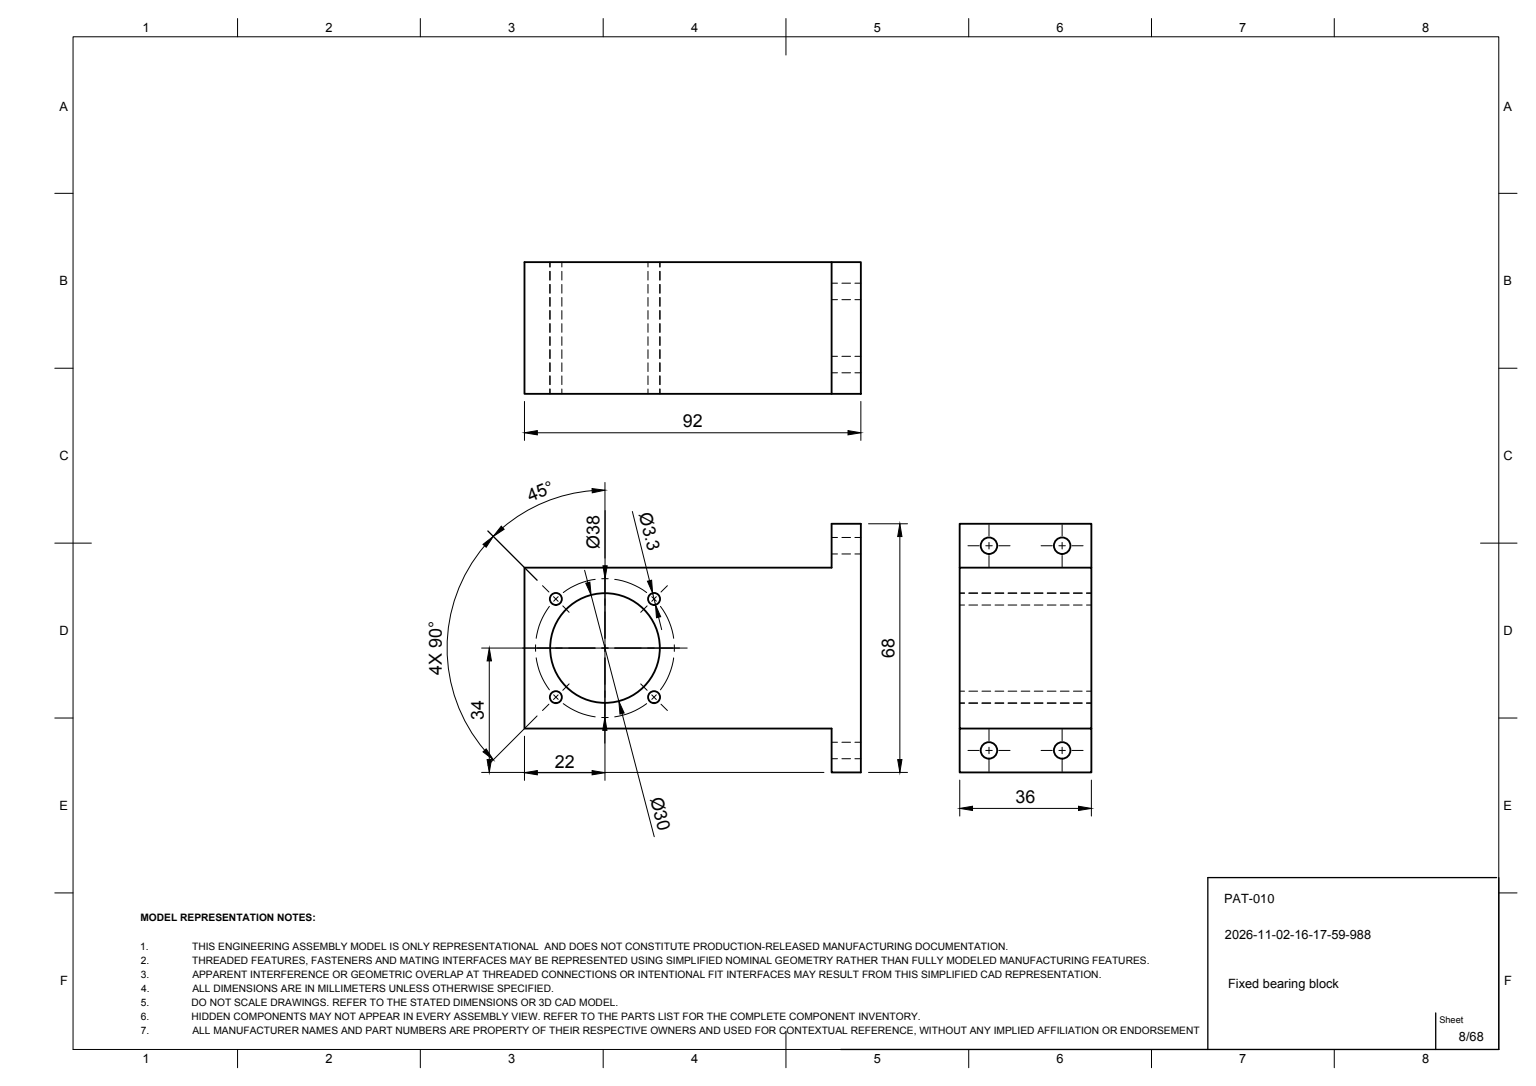
ISO-10303-21;
HEADER;
/* Generated by software containing ST-Developer
 * from STEP Tools, Inc. (www.steptools.com) 
 */

FILE_DESCRIPTION(
/* description */ ('Belt conveyor head drive unit'),
/* implementation_level */ '2;1');

FILE_NAME(
/* name */ 'Fixed bearing block.step',
/* time_stamp */ '2026-10-28T03:26:19-07:00',
/* author */ (''),
/* organization */ (''),
/* preprocessor_version */ 'ST-DEVELOPER v20.2',
/* originating_system */ 'Autodesk Translation Framework v15.17.0.0',
/* authorisation */ '');

FILE_SCHEMA (('AUTOMOTIVE_DESIGN { 1 0 10303 214 3 1 1 }'));
ENDSEC;

DATA;
#10=MECHANICAL_DESIGN_GEOMETRIC_PRESENTATION_REPRESENTATION('',(#850),#27069);
#712=SHAPE_REPRESENTATION_RELATIONSHIP('SRR','None',#27356,#781);
#781=ADVANCED_BREP_SHAPE_REPRESENTATION('',(#935),#26998);
#850=STYLED_ITEM('',(#27797),#935);
#935=MANIFOLD_SOLID_BREP('Body1',#13715);
#1032=FACE_BOUND('',#2525,.T.);
#1033=FACE_BOUND('',#2526,.T.);
#1034=FACE_BOUND('',#2528,.T.);
#1035=FACE_BOUND('',#2529,.T.);
#1036=FACE_BOUND('',#2533,.T.);
#1037=FACE_BOUND('',#2534,.T.);
#1038=FACE_BOUND('',#2535,.T.);
#1039=FACE_BOUND('',#2536,.T.);
#1040=FACE_BOUND('',#2537,.T.);
#1041=FACE_BOUND('',#2540,.T.);
#1042=FACE_BOUND('',#2541,.T.);
#1043=FACE_BOUND('',#2542,.T.);
#1044=FACE_BOUND('',#2543,.T.);
#1045=FACE_BOUND('',#2544,.T.);
#1046=FACE_BOUND('',#2548,.T.);
#1047=FACE_BOUND('',#2549,.T.);
#1048=FACE_BOUND('',#2550,.T.);
#1049=FACE_BOUND('',#2551,.T.);
#1317=PLANE('',#14705);
#1318=PLANE('',#14706);
#1319=PLANE('',#14707);
#1320=PLANE('',#14708);
#1321=PLANE('',#14709);
#1322=PLANE('',#14710);
#1323=PLANE('',#14711);
#1324=PLANE('',#14712);
#1325=PLANE('',#14713);
#1326=PLANE('',#14714);
#1695=FACE_OUTER_BOUND('',#2515,.T.);
#1696=FACE_OUTER_BOUND('',#2516,.T.);
#1697=FACE_OUTER_BOUND('',#2517,.T.);
#1698=FACE_OUTER_BOUND('',#2518,.T.);
#1699=FACE_OUTER_BOUND('',#2519,.T.);
#1700=FACE_OUTER_BOUND('',#2520,.T.);
#1701=FACE_OUTER_BOUND('',#2521,.T.);
#1702=FACE_OUTER_BOUND('',#2522,.T.);
#1703=FACE_OUTER_BOUND('',#2523,.T.);
#1704=FACE_OUTER_BOUND('',#2524,.T.);
#1705=FACE_OUTER_BOUND('',#2527,.T.);
#1706=FACE_OUTER_BOUND('',#2530,.T.);
#1707=FACE_OUTER_BOUND('',#2531,.T.);
#1708=FACE_OUTER_BOUND('',#2532,.T.);
#1709=FACE_OUTER_BOUND('',#2538,.T.);
#1710=FACE_OUTER_BOUND('',#2539,.T.);
#1711=FACE_OUTER_BOUND('',#2545,.T.);
#1712=FACE_OUTER_BOUND('',#2546,.T.);
#1713=FACE_OUTER_BOUND('',#2547,.T.);
#2515=EDGE_LOOP('',(#9222,#9223,#9224,#9225));
#2516=EDGE_LOOP('',(#9226,#9227,#9228,#9229));
#2517=EDGE_LOOP('',(#9230,#9231,#9232,#9233));
#2518=EDGE_LOOP('',(#9234,#9235,#9236,#9237));
#2519=EDGE_LOOP('',(#9238,#9239,#9240,#9241));
#2520=EDGE_LOOP('',(#9242,#9243,#9244,#9245));
#2521=EDGE_LOOP('',(#9246,#9247,#9248,#9249));
#2522=EDGE_LOOP('',(#9250,#9251,#9252,#9253));
#2523=EDGE_LOOP('',(#9254,#9255,#9256,#9257));
#2524=EDGE_LOOP('',(#9258,#9259,#9260,#9261));
#2525=EDGE_LOOP('',(#9262));
#2526=EDGE_LOOP('',(#9263));
#2527=EDGE_LOOP('',(#9264,#9265,#9266,#9267));
#2528=EDGE_LOOP('',(#9268));
#2529=EDGE_LOOP('',(#9269));
#2530=EDGE_LOOP('',(#9270,#9271,#9272,#9273));
#2531=EDGE_LOOP('',(#9274,#9275,#9276,#9277));
#2532=EDGE_LOOP('',(#9278,#9279,#9280,#9281,#9282,#9283,#9284,#9285));
#2533=EDGE_LOOP('',(#9286));
#2534=EDGE_LOOP('',(#9287));
#2535=EDGE_LOOP('',(#9288));
#2536=EDGE_LOOP('',(#9289));
#2537=EDGE_LOOP('',(#9290));
#2538=EDGE_LOOP('',(#9291,#9292,#9293,#9294));
#2539=EDGE_LOOP('',(#9295,#9296,#9297,#9298,#9299,#9300,#9301,#9302));
#2540=EDGE_LOOP('',(#9303));
#2541=EDGE_LOOP('',(#9304));
#2542=EDGE_LOOP('',(#9305));
#2543=EDGE_LOOP('',(#9306));
#2544=EDGE_LOOP('',(#9307));
#2545=EDGE_LOOP('',(#9308,#9309,#9310,#9311));
#2546=EDGE_LOOP('',(#9312,#9313,#9314,#9315));
#2547=EDGE_LOOP('',(#9316,#9317,#9318,#9319));
#2548=EDGE_LOOP('',(#9320));
#2549=EDGE_LOOP('',(#9321));
#2550=EDGE_LOOP('',(#9322));
#2551=EDGE_LOOP('',(#9323));
#3582=LINE('',#21262,#4374);
#3583=LINE('',#21268,#4375);
#3584=LINE('',#21274,#4376);
#3585=LINE('',#21280,#4377);
#3586=LINE('',#21286,#4378);
#3587=LINE('',#21292,#4379);
#3588=LINE('',#21298,#4380);
#3589=LINE('',#21304,#4381);
#3590=LINE('',#21310,#4382);
#3591=LINE('',#21315,#4383);
#3592=LINE('',#21317,#4384);
#3593=LINE('',#21319,#4385);
#3594=LINE('',#21320,#4386);
#3595=LINE('',#21324,#4387);
#3596=LINE('',#21326,#4388);
#3597=LINE('',#21328,#4389);
#3598=LINE('',#21329,#4390);
#3599=LINE('',#21332,#4391);
#3600=LINE('',#21334,#4392);
#3601=LINE('',#21335,#4393);
#3602=LINE('',#21338,#4394);
#3603=LINE('',#21340,#4395);
#3604=LINE('',#21341,#4396);
#3605=LINE('',#21344,#4397);
#3606=LINE('',#21346,#4398);
#3607=LINE('',#21347,#4399);
#3608=LINE('',#21348,#4400);
#3609=LINE('',#21351,#4401);
#3610=LINE('',#21352,#4402);
#3611=LINE('',#21355,#4403);
#3612=LINE('',#21356,#4404);
#3613=LINE('',#21357,#4405);
#3614=LINE('',#21359,#4406);
#4374=VECTOR('',#16754,0.165);
#4375=VECTOR('',#16761,0.165);
#4376=VECTOR('',#16768,0.165);
#4377=VECTOR('',#16775,0.165);
#4378=VECTOR('',#16782,1.5);
#4379=VECTOR('',#16789,0.225);
#4380=VECTOR('',#16796,0.225);
#4381=VECTOR('',#16803,0.225);
#4382=VECTOR('',#16810,0.225);
#4383=VECTOR('',#16815,1.);
#4384=VECTOR('',#16816,1.);
#4385=VECTOR('',#16817,1.);
#4386=VECTOR('',#16818,1.);
#4387=VECTOR('',#16821,1.);
#4388=VECTOR('',#16822,1.);
#4389=VECTOR('',#16823,1.);
#4390=VECTOR('',#16824,1.);
#4391=VECTOR('',#16827,1.);
#4392=VECTOR('',#16828,1.);
#4393=VECTOR('',#16829,1.);
#4394=VECTOR('',#16832,1.);
#4395=VECTOR('',#16833,1.);
#4396=VECTOR('',#16834,1.);
#4397=VECTOR('',#16837,1.);
#4398=VECTOR('',#16838,1.);
#4399=VECTOR('',#16839,1.);
#4400=VECTOR('',#16840,1.);
#4401=VECTOR('',#16843,1.);
#4402=VECTOR('',#16844,1.);
#4403=VECTOR('',#16847,1.);
#4404=VECTOR('',#16848,1.);
#4405=VECTOR('',#16849,1.);
#4406=VECTOR('',#16852,1.);
#5130=CIRCLE('',#14679,0.165);
#5131=CIRCLE('',#14680,0.165);
#5132=CIRCLE('',#14682,0.165);
#5133=CIRCLE('',#14683,0.165);
#5134=CIRCLE('',#14685,0.165);
#5135=CIRCLE('',#14686,0.165);
#5136=CIRCLE('',#14688,0.165);
#5137=CIRCLE('',#14689,0.165);
#5138=CIRCLE('',#14691,1.5);
#5139=CIRCLE('',#14692,1.5);
#5140=CIRCLE('',#14694,0.225);
#5141=CIRCLE('',#14695,0.225);
#5142=CIRCLE('',#14697,0.225);
#5143=CIRCLE('',#14698,0.225);
#5144=CIRCLE('',#14700,0.225);
#5145=CIRCLE('',#14701,0.225);
#5146=CIRCLE('',#14703,0.225);
#5147=CIRCLE('',#14704,0.225);
#6041=VERTEX_POINT('',#21259);
#6042=VERTEX_POINT('',#21261);
#6043=VERTEX_POINT('',#21265);
#6044=VERTEX_POINT('',#21267);
#6045=VERTEX_POINT('',#21271);
#6046=VERTEX_POINT('',#21273);
#6047=VERTEX_POINT('',#21277);
#6048=VERTEX_POINT('',#21279);
#6049=VERTEX_POINT('',#21283);
#6050=VERTEX_POINT('',#21285);
#6051=VERTEX_POINT('',#21289);
#6052=VERTEX_POINT('',#21291);
#6053=VERTEX_POINT('',#21295);
#6054=VERTEX_POINT('',#21297);
#6055=VERTEX_POINT('',#21301);
#6056=VERTEX_POINT('',#21303);
#6057=VERTEX_POINT('',#21307);
#6058=VERTEX_POINT('',#21309);
#6059=VERTEX_POINT('',#21313);
#6060=VERTEX_POINT('',#21314);
#6061=VERTEX_POINT('',#21316);
#6062=VERTEX_POINT('',#21318);
#6063=VERTEX_POINT('',#21322);
#6064=VERTEX_POINT('',#21323);
#6065=VERTEX_POINT('',#21325);
#6066=VERTEX_POINT('',#21327);
#6067=VERTEX_POINT('',#21331);
#6068=VERTEX_POINT('',#21333);
#6069=VERTEX_POINT('',#21337);
#6070=VERTEX_POINT('',#21339);
#6071=VERTEX_POINT('',#21343);
#6072=VERTEX_POINT('',#21345);
#6073=VERTEX_POINT('',#21350);
#6074=VERTEX_POINT('',#21354);
#7303=EDGE_CURVE('',#6041,#6041,#5130,.T.);
#7304=EDGE_CURVE('',#6041,#6042,#3582,.T.);
#7305=EDGE_CURVE('',#6042,#6042,#5131,.T.);
#7306=EDGE_CURVE('',#6043,#6043,#5132,.T.);
#7307=EDGE_CURVE('',#6043,#6044,#3583,.T.);
#7308=EDGE_CURVE('',#6044,#6044,#5133,.T.);
#7309=EDGE_CURVE('',#6045,#6045,#5134,.T.);
#7310=EDGE_CURVE('',#6045,#6046,#3584,.T.);
#7311=EDGE_CURVE('',#6046,#6046,#5135,.T.);
#7312=EDGE_CURVE('',#6047,#6047,#5136,.T.);
#7313=EDGE_CURVE('',#6047,#6048,#3585,.T.);
#7314=EDGE_CURVE('',#6048,#6048,#5137,.T.);
#7315=EDGE_CURVE('',#6049,#6049,#5138,.T.);
#7316=EDGE_CURVE('',#6049,#6050,#3586,.T.);
#7317=EDGE_CURVE('',#6050,#6050,#5139,.T.);
#7318=EDGE_CURVE('',#6051,#6051,#5140,.T.);
#7319=EDGE_CURVE('',#6051,#6052,#3587,.T.);
#7320=EDGE_CURVE('',#6052,#6052,#5141,.T.);
#7321=EDGE_CURVE('',#6053,#6053,#5142,.T.);
#7322=EDGE_CURVE('',#6053,#6054,#3588,.T.);
#7323=EDGE_CURVE('',#6054,#6054,#5143,.T.);
#7324=EDGE_CURVE('',#6055,#6055,#5144,.T.);
#7325=EDGE_CURVE('',#6055,#6056,#3589,.T.);
#7326=EDGE_CURVE('',#6056,#6056,#5145,.T.);
#7327=EDGE_CURVE('',#6057,#6057,#5146,.T.);
#7328=EDGE_CURVE('',#6057,#6058,#3590,.T.);
#7329=EDGE_CURVE('',#6058,#6058,#5147,.T.);
#7330=EDGE_CURVE('',#6059,#6060,#3591,.T.);
#7331=EDGE_CURVE('',#6061,#6059,#3592,.T.);
#7332=EDGE_CURVE('',#6061,#6062,#3593,.T.);
#7333=EDGE_CURVE('',#6060,#6062,#3594,.T.);
#7334=EDGE_CURVE('',#6063,#6064,#3595,.T.);
#7335=EDGE_CURVE('',#6065,#6063,#3596,.T.);
#7336=EDGE_CURVE('',#6066,#6065,#3597,.T.);
#7337=EDGE_CURVE('',#6064,#6066,#3598,.T.);
#7338=EDGE_CURVE('',#6066,#6067,#3599,.T.);
#7339=EDGE_CURVE('',#6068,#6065,#3600,.T.);
#7340=EDGE_CURVE('',#6067,#6068,#3601,.T.);
#7341=EDGE_CURVE('',#6069,#6061,#3602,.T.);
#7342=EDGE_CURVE('',#6069,#6070,#3603,.T.);
#7343=EDGE_CURVE('',#6062,#6070,#3604,.T.);
#7344=EDGE_CURVE('',#6059,#6071,#3605,.T.);
#7345=EDGE_CURVE('',#6072,#6071,#3606,.T.);
#7346=EDGE_CURVE('',#6064,#6072,#3607,.T.);
#7347=EDGE_CURVE('',#6067,#6069,#3608,.T.);
#7348=EDGE_CURVE('',#6060,#6073,#3609,.T.);
#7349=EDGE_CURVE('',#6071,#6073,#3610,.T.);
#7350=EDGE_CURVE('',#6063,#6074,#3611,.T.);
#7351=EDGE_CURVE('',#6073,#6074,#3612,.T.);
#7352=EDGE_CURVE('',#6070,#6068,#3613,.T.);
#7353=EDGE_CURVE('',#6074,#6072,#3614,.T.);
#9222=ORIENTED_EDGE('',*,*,#7303,.F.);
#9223=ORIENTED_EDGE('',*,*,#7304,.T.);
#9224=ORIENTED_EDGE('',*,*,#7305,.F.);
#9225=ORIENTED_EDGE('',*,*,#7304,.F.);
#9226=ORIENTED_EDGE('',*,*,#7306,.F.);
#9227=ORIENTED_EDGE('',*,*,#7307,.T.);
#9228=ORIENTED_EDGE('',*,*,#7308,.F.);
#9229=ORIENTED_EDGE('',*,*,#7307,.F.);
#9230=ORIENTED_EDGE('',*,*,#7309,.F.);
#9231=ORIENTED_EDGE('',*,*,#7310,.T.);
#9232=ORIENTED_EDGE('',*,*,#7311,.F.);
#9233=ORIENTED_EDGE('',*,*,#7310,.F.);
#9234=ORIENTED_EDGE('',*,*,#7312,.F.);
#9235=ORIENTED_EDGE('',*,*,#7313,.T.);
#9236=ORIENTED_EDGE('',*,*,#7314,.F.);
#9237=ORIENTED_EDGE('',*,*,#7313,.F.);
#9238=ORIENTED_EDGE('',*,*,#7315,.F.);
#9239=ORIENTED_EDGE('',*,*,#7316,.T.);
#9240=ORIENTED_EDGE('',*,*,#7317,.F.);
#9241=ORIENTED_EDGE('',*,*,#7316,.F.);
#9242=ORIENTED_EDGE('',*,*,#7318,.F.);
#9243=ORIENTED_EDGE('',*,*,#7319,.T.);
#9244=ORIENTED_EDGE('',*,*,#7320,.F.);
#9245=ORIENTED_EDGE('',*,*,#7319,.F.);
#9246=ORIENTED_EDGE('',*,*,#7321,.F.);
#9247=ORIENTED_EDGE('',*,*,#7322,.T.);
#9248=ORIENTED_EDGE('',*,*,#7323,.F.);
#9249=ORIENTED_EDGE('',*,*,#7322,.F.);
#9250=ORIENTED_EDGE('',*,*,#7324,.F.);
#9251=ORIENTED_EDGE('',*,*,#7325,.T.);
#9252=ORIENTED_EDGE('',*,*,#7326,.F.);
#9253=ORIENTED_EDGE('',*,*,#7325,.F.);
#9254=ORIENTED_EDGE('',*,*,#7327,.F.);
#9255=ORIENTED_EDGE('',*,*,#7328,.T.);
#9256=ORIENTED_EDGE('',*,*,#7329,.F.);
#9257=ORIENTED_EDGE('',*,*,#7328,.F.);
#9258=ORIENTED_EDGE('',*,*,#7330,.F.);
#9259=ORIENTED_EDGE('',*,*,#7331,.F.);
#9260=ORIENTED_EDGE('',*,*,#7332,.T.);
#9261=ORIENTED_EDGE('',*,*,#7333,.F.);
#9262=ORIENTED_EDGE('',*,*,#7320,.T.);
#9263=ORIENTED_EDGE('',*,*,#7329,.T.);
#9264=ORIENTED_EDGE('',*,*,#7334,.F.);
#9265=ORIENTED_EDGE('',*,*,#7335,.F.);
#9266=ORIENTED_EDGE('',*,*,#7336,.F.);
#9267=ORIENTED_EDGE('',*,*,#7337,.F.);
#9268=ORIENTED_EDGE('',*,*,#7323,.T.);
#9269=ORIENTED_EDGE('',*,*,#7326,.T.);
#9270=ORIENTED_EDGE('',*,*,#7338,.F.);
#9271=ORIENTED_EDGE('',*,*,#7336,.T.);
#9272=ORIENTED_EDGE('',*,*,#7339,.F.);
#9273=ORIENTED_EDGE('',*,*,#7340,.F.);
#9274=ORIENTED_EDGE('',*,*,#7341,.F.);
#9275=ORIENTED_EDGE('',*,*,#7342,.T.);
#9276=ORIENTED_EDGE('',*,*,#7343,.F.);
#9277=ORIENTED_EDGE('',*,*,#7332,.F.);
#9278=ORIENTED_EDGE('',*,*,#7344,.T.);
#9279=ORIENTED_EDGE('',*,*,#7345,.F.);
#9280=ORIENTED_EDGE('',*,*,#7346,.F.);
#9281=ORIENTED_EDGE('',*,*,#7337,.T.);
#9282=ORIENTED_EDGE('',*,*,#7338,.T.);
#9283=ORIENTED_EDGE('',*,*,#7347,.T.);
#9284=ORIENTED_EDGE('',*,*,#7341,.T.);
#9285=ORIENTED_EDGE('',*,*,#7331,.T.);
#9286=ORIENTED_EDGE('',*,*,#7315,.T.);
#9287=ORIENTED_EDGE('',*,*,#7312,.T.);
#9288=ORIENTED_EDGE('',*,*,#7309,.T.);
#9289=ORIENTED_EDGE('',*,*,#7306,.T.);
#9290=ORIENTED_EDGE('',*,*,#7303,.T.);
#9291=ORIENTED_EDGE('',*,*,#7330,.T.);
#9292=ORIENTED_EDGE('',*,*,#7348,.T.);
#9293=ORIENTED_EDGE('',*,*,#7349,.F.);
#9294=ORIENTED_EDGE('',*,*,#7344,.F.);
#9295=ORIENTED_EDGE('',*,*,#7350,.T.);
#9296=ORIENTED_EDGE('',*,*,#7351,.F.);
#9297=ORIENTED_EDGE('',*,*,#7348,.F.);
#9298=ORIENTED_EDGE('',*,*,#7333,.T.);
#9299=ORIENTED_EDGE('',*,*,#7343,.T.);
#9300=ORIENTED_EDGE('',*,*,#7352,.T.);
#9301=ORIENTED_EDGE('',*,*,#7339,.T.);
#9302=ORIENTED_EDGE('',*,*,#7335,.T.);
#9303=ORIENTED_EDGE('',*,*,#7317,.T.);
#9304=ORIENTED_EDGE('',*,*,#7314,.T.);
#9305=ORIENTED_EDGE('',*,*,#7311,.T.);
#9306=ORIENTED_EDGE('',*,*,#7308,.T.);
#9307=ORIENTED_EDGE('',*,*,#7305,.T.);
#9308=ORIENTED_EDGE('',*,*,#7334,.T.);
#9309=ORIENTED_EDGE('',*,*,#7346,.T.);
#9310=ORIENTED_EDGE('',*,*,#7353,.F.);
#9311=ORIENTED_EDGE('',*,*,#7350,.F.);
#9312=ORIENTED_EDGE('',*,*,#7353,.T.);
#9313=ORIENTED_EDGE('',*,*,#7345,.T.);
#9314=ORIENTED_EDGE('',*,*,#7349,.T.);
#9315=ORIENTED_EDGE('',*,*,#7351,.T.);
#9316=ORIENTED_EDGE('',*,*,#7352,.F.);
#9317=ORIENTED_EDGE('',*,*,#7342,.F.);
#9318=ORIENTED_EDGE('',*,*,#7347,.F.);
#9319=ORIENTED_EDGE('',*,*,#7340,.T.);
#9320=ORIENTED_EDGE('',*,*,#7318,.T.);
#9321=ORIENTED_EDGE('',*,*,#7321,.T.);
#9322=ORIENTED_EDGE('',*,*,#7324,.T.);
#9323=ORIENTED_EDGE('',*,*,#7327,.T.);
#12554=CYLINDRICAL_SURFACE('',#14678,0.165);
#12555=CYLINDRICAL_SURFACE('',#14681,0.165);
#12556=CYLINDRICAL_SURFACE('',#14684,0.165);
#12557=CYLINDRICAL_SURFACE('',#14687,0.165);
#12558=CYLINDRICAL_SURFACE('',#14690,1.5);
#12559=CYLINDRICAL_SURFACE('',#14693,0.225);
#12560=CYLINDRICAL_SURFACE('',#14696,0.225);
#12561=CYLINDRICAL_SURFACE('',#14699,0.225);
#12562=CYLINDRICAL_SURFACE('',#14702,0.225);
#12974=ADVANCED_FACE('',(#1695),#12554,.F.);
#12975=ADVANCED_FACE('',(#1696),#12555,.F.);
#12976=ADVANCED_FACE('',(#1697),#12556,.F.);
#12977=ADVANCED_FACE('',(#1698),#12557,.F.);
#12978=ADVANCED_FACE('',(#1699),#12558,.F.);
#12979=ADVANCED_FACE('',(#1700),#12559,.F.);
#12980=ADVANCED_FACE('',(#1701),#12560,.F.);
#12981=ADVANCED_FACE('',(#1702),#12561,.F.);
#12982=ADVANCED_FACE('',(#1703),#12562,.F.);
#12983=ADVANCED_FACE('',(#1704,#1032,#1033),#1317,.T.);
#12984=ADVANCED_FACE('',(#1705,#1034,#1035),#1318,.T.);
#12985=ADVANCED_FACE('',(#1706),#1319,.T.);
#12986=ADVANCED_FACE('',(#1707),#1320,.T.);
#12987=ADVANCED_FACE('',(#1708,#1036,#1037,#1038,#1039,#1040),#1321,.T.);
#12988=ADVANCED_FACE('',(#1709),#1322,.T.);
#12989=ADVANCED_FACE('',(#1710,#1041,#1042,#1043,#1044,#1045),#1323,.T.);
#12990=ADVANCED_FACE('',(#1711),#1324,.T.);
#12991=ADVANCED_FACE('',(#1712),#1325,.T.);
#12992=ADVANCED_FACE('',(#1713,#1046,#1047,#1048,#1049),#1326,.F.);
#13715=CLOSED_SHELL('',(#12974,#12975,#12976,#12977,#12978,#12979,#12980,
#12981,#12982,#12983,#12984,#12985,#12986,#12987,#12988,#12989,#12990,#12991,
#12992));
#14677=AXIS2_PLACEMENT_3D('',#21257,#16748,#16749);
#14678=AXIS2_PLACEMENT_3D('',#21258,#16750,#16751);
#14679=AXIS2_PLACEMENT_3D('',#21260,#16752,#16753);
#14680=AXIS2_PLACEMENT_3D('',#21263,#16755,#16756);
#14681=AXIS2_PLACEMENT_3D('',#21264,#16757,#16758);
#14682=AXIS2_PLACEMENT_3D('',#21266,#16759,#16760);
#14683=AXIS2_PLACEMENT_3D('',#21269,#16762,#16763);
#14684=AXIS2_PLACEMENT_3D('',#21270,#16764,#16765);
#14685=AXIS2_PLACEMENT_3D('',#21272,#16766,#16767);
#14686=AXIS2_PLACEMENT_3D('',#21275,#16769,#16770);
#14687=AXIS2_PLACEMENT_3D('',#21276,#16771,#16772);
#14688=AXIS2_PLACEMENT_3D('',#21278,#16773,#16774);
#14689=AXIS2_PLACEMENT_3D('',#21281,#16776,#16777);
#14690=AXIS2_PLACEMENT_3D('',#21282,#16778,#16779);
#14691=AXIS2_PLACEMENT_3D('',#21284,#16780,#16781);
#14692=AXIS2_PLACEMENT_3D('',#21287,#16783,#16784);
#14693=AXIS2_PLACEMENT_3D('',#21288,#16785,#16786);
#14694=AXIS2_PLACEMENT_3D('',#21290,#16787,#16788);
#14695=AXIS2_PLACEMENT_3D('',#21293,#16790,#16791);
#14696=AXIS2_PLACEMENT_3D('',#21294,#16792,#16793);
#14697=AXIS2_PLACEMENT_3D('',#21296,#16794,#16795);
#14698=AXIS2_PLACEMENT_3D('',#21299,#16797,#16798);
#14699=AXIS2_PLACEMENT_3D('',#21300,#16799,#16800);
#14700=AXIS2_PLACEMENT_3D('',#21302,#16801,#16802);
#14701=AXIS2_PLACEMENT_3D('',#21305,#16804,#16805);
#14702=AXIS2_PLACEMENT_3D('',#21306,#16806,#16807);
#14703=AXIS2_PLACEMENT_3D('',#21308,#16808,#16809);
#14704=AXIS2_PLACEMENT_3D('',#21311,#16811,#16812);
#14705=AXIS2_PLACEMENT_3D('',#21312,#16813,#16814);
#14706=AXIS2_PLACEMENT_3D('',#21321,#16819,#16820);
#14707=AXIS2_PLACEMENT_3D('',#21330,#16825,#16826);
#14708=AXIS2_PLACEMENT_3D('',#21336,#16830,#16831);
#14709=AXIS2_PLACEMENT_3D('',#21342,#16835,#16836);
#14710=AXIS2_PLACEMENT_3D('',#21349,#16841,#16842);
#14711=AXIS2_PLACEMENT_3D('',#21353,#16845,#16846);
#14712=AXIS2_PLACEMENT_3D('',#21358,#16850,#16851);
#14713=AXIS2_PLACEMENT_3D('',#21360,#16853,#16854);
#14714=AXIS2_PLACEMENT_3D('',#21361,#16855,#16856);
#16748=DIRECTION('axis',(0.,0.,1.));
#16749=DIRECTION('refdir',(1.,0.,0.));
#16750=DIRECTION('center_axis',(0.,1.,0.));
#16751=DIRECTION('ref_axis',(1.,0.,0.));
#16752=DIRECTION('center_axis',(0.,1.,0.));
#16753=DIRECTION('ref_axis',(1.,0.,0.));
#16754=DIRECTION('',(0.,1.,0.));
#16755=DIRECTION('center_axis',(0.,-1.,0.));
#16756=DIRECTION('ref_axis',(1.,0.,0.));
#16757=DIRECTION('center_axis',(0.,1.,0.));
#16758=DIRECTION('ref_axis',(1.,0.,0.));
#16759=DIRECTION('center_axis',(0.,1.,0.));
#16760=DIRECTION('ref_axis',(1.,0.,0.));
#16761=DIRECTION('',(0.,1.,0.));
#16762=DIRECTION('center_axis',(0.,-1.,0.));
#16763=DIRECTION('ref_axis',(1.,0.,0.));
#16764=DIRECTION('center_axis',(0.,1.,0.));
#16765=DIRECTION('ref_axis',(1.,0.,0.));
#16766=DIRECTION('center_axis',(0.,1.,0.));
#16767=DIRECTION('ref_axis',(1.,0.,0.));
#16768=DIRECTION('',(0.,1.,0.));
#16769=DIRECTION('center_axis',(0.,-1.,0.));
#16770=DIRECTION('ref_axis',(1.,0.,0.));
#16771=DIRECTION('center_axis',(0.,1.,0.));
#16772=DIRECTION('ref_axis',(1.,0.,0.));
#16773=DIRECTION('center_axis',(0.,1.,0.));
#16774=DIRECTION('ref_axis',(1.,0.,0.));
#16775=DIRECTION('',(0.,1.,0.));
#16776=DIRECTION('center_axis',(0.,-1.,0.));
#16777=DIRECTION('ref_axis',(1.,0.,0.));
#16778=DIRECTION('center_axis',(0.,1.,0.));
#16779=DIRECTION('ref_axis',(1.,0.,0.));
#16780=DIRECTION('center_axis',(0.,1.,0.));
#16781=DIRECTION('ref_axis',(1.,0.,0.));
#16782=DIRECTION('',(0.,1.,0.));
#16783=DIRECTION('center_axis',(0.,-1.,0.));
#16784=DIRECTION('ref_axis',(1.,0.,0.));
#16785=DIRECTION('center_axis',(0.,0.,1.));
#16786=DIRECTION('ref_axis',(1.,0.,0.));
#16787=DIRECTION('center_axis',(0.,0.,1.));
#16788=DIRECTION('ref_axis',(1.,0.,0.));
#16789=DIRECTION('',(0.,0.,1.));
#16790=DIRECTION('center_axis',(0.,0.,-1.));
#16791=DIRECTION('ref_axis',(1.,0.,0.));
#16792=DIRECTION('center_axis',(0.,0.,1.));
#16793=DIRECTION('ref_axis',(1.,0.,0.));
#16794=DIRECTION('center_axis',(0.,0.,1.));
#16795=DIRECTION('ref_axis',(1.,0.,0.));
#16796=DIRECTION('',(0.,0.,1.));
#16797=DIRECTION('center_axis',(0.,0.,-1.));
#16798=DIRECTION('ref_axis',(1.,0.,0.));
#16799=DIRECTION('center_axis',(0.,0.,1.));
#16800=DIRECTION('ref_axis',(1.,0.,0.));
#16801=DIRECTION('center_axis',(0.,0.,1.));
#16802=DIRECTION('ref_axis',(1.,0.,0.));
#16803=DIRECTION('',(0.,0.,1.));
#16804=DIRECTION('center_axis',(0.,0.,-1.));
#16805=DIRECTION('ref_axis',(1.,0.,0.));
#16806=DIRECTION('center_axis',(0.,0.,1.));
#16807=DIRECTION('ref_axis',(1.,0.,0.));
#16808=DIRECTION('center_axis',(0.,0.,1.));
#16809=DIRECTION('ref_axis',(1.,0.,0.));
#16810=DIRECTION('',(0.,0.,1.));
#16811=DIRECTION('center_axis',(0.,0.,-1.));
#16812=DIRECTION('ref_axis',(1.,0.,0.));
#16813=DIRECTION('center_axis',(0.,0.,1.));
#16814=DIRECTION('ref_axis',(1.,0.,0.));
#16815=DIRECTION('',(0.,1.,0.));
#16816=DIRECTION('',(-1.,0.,0.));
#16817=DIRECTION('',(0.,1.,0.));
#16818=DIRECTION('',(1.,0.,0.));
#16819=DIRECTION('center_axis',(0.,0.,1.));
#16820=DIRECTION('ref_axis',(1.,0.,0.));
#16821=DIRECTION('',(0.,-1.,0.));
#16822=DIRECTION('',(1.,0.,0.));
#16823=DIRECTION('',(0.,1.,0.));
#16824=DIRECTION('',(-1.,0.,0.));
#16825=DIRECTION('center_axis',(-1.,0.,0.));
#16826=DIRECTION('ref_axis',(0.,0.,1.));
#16827=DIRECTION('',(0.,0.,-1.));
#16828=DIRECTION('',(0.,0.,1.));
#16829=DIRECTION('',(0.,1.,0.));
#16830=DIRECTION('center_axis',(1.,0.,0.));
#16831=DIRECTION('ref_axis',(0.,0.,-1.));
#16832=DIRECTION('',(0.,0.,1.));
#16833=DIRECTION('',(0.,1.,0.));
#16834=DIRECTION('',(0.,0.,-1.));
#16835=DIRECTION('center_axis',(0.,-1.,0.));
#16836=DIRECTION('ref_axis',(1.,0.,0.));
#16837=DIRECTION('',(0.,0.,1.));
#16838=DIRECTION('',(1.,0.,0.));
#16839=DIRECTION('',(0.,0.,1.));
#16840=DIRECTION('',(1.,0.,0.));
#16841=DIRECTION('center_axis',(1.,0.,0.));
#16842=DIRECTION('ref_axis',(0.,1.,0.));
#16843=DIRECTION('',(0.,0.,1.));
#16844=DIRECTION('',(0.,1.,0.));
#16845=DIRECTION('center_axis',(0.,1.,0.));
#16846=DIRECTION('ref_axis',(-1.,0.,0.));
#16847=DIRECTION('',(0.,0.,1.));
#16848=DIRECTION('',(-1.,0.,0.));
#16849=DIRECTION('',(-1.,0.,0.));
#16850=DIRECTION('center_axis',(-1.,0.,0.));
#16851=DIRECTION('ref_axis',(0.,-1.,0.));
#16852=DIRECTION('',(0.,-1.,0.));
#16853=DIRECTION('center_axis',(0.,0.,1.));
#16854=DIRECTION('ref_axis',(1.,0.,0.));
#16855=DIRECTION('center_axis',(0.,0.,1.));
#16856=DIRECTION('ref_axis',(1.,0.,0.));
#21257=CARTESIAN_POINT('',(0.,0.,0.));
#21258=CARTESIAN_POINT('Origin',(-1.34350288425444,-1.9,5.65649711574556));
#21259=CARTESIAN_POINT('',(-1.50850288425444,-1.8,5.65649711574556));
#21260=CARTESIAN_POINT('Origin',(-1.34350288425444,-1.8,5.65649711574556));
#21261=CARTESIAN_POINT('',(-1.50850288425444,1.8,5.65649711574556));
#21262=CARTESIAN_POINT('',(-1.50850288425444,-1.9,5.65649711574556));
#21263=CARTESIAN_POINT('Origin',(-1.34350288425444,1.8,5.65649711574556));
#21264=CARTESIAN_POINT('Origin',(-1.34350288425444,-1.9,8.34350288425444));
#21265=CARTESIAN_POINT('',(-1.50850288425444,-1.8,8.34350288425444));
#21266=CARTESIAN_POINT('Origin',(-1.34350288425444,-1.8,8.34350288425444));
#21267=CARTESIAN_POINT('',(-1.50850288425444,1.8,8.34350288425444));
#21268=CARTESIAN_POINT('',(-1.50850288425444,-1.9,8.34350288425444));
#21269=CARTESIAN_POINT('Origin',(-1.34350288425444,1.8,8.34350288425444));
#21270=CARTESIAN_POINT('Origin',(1.34350288425444,-1.9,8.34350288425444));
#21271=CARTESIAN_POINT('',(1.17850288425444,-1.8,8.34350288425444));
#21272=CARTESIAN_POINT('Origin',(1.34350288425444,-1.8,8.34350288425444));
#21273=CARTESIAN_POINT('',(1.17850288425444,1.8,8.34350288425444));
#21274=CARTESIAN_POINT('',(1.17850288425444,-1.9,8.34350288425444));
#21275=CARTESIAN_POINT('Origin',(1.34350288425444,1.8,8.34350288425444));
#21276=CARTESIAN_POINT('Origin',(1.34350288425444,-1.9,5.65649711574556));
#21277=CARTESIAN_POINT('',(1.17850288425444,-1.8,5.65649711574556));
#21278=CARTESIAN_POINT('Origin',(1.34350288425444,-1.8,5.65649711574556));
#21279=CARTESIAN_POINT('',(1.17850288425444,1.8,5.65649711574556));
#21280=CARTESIAN_POINT('',(1.17850288425444,-1.9,5.65649711574556));
#21281=CARTESIAN_POINT('Origin',(1.34350288425444,1.8,5.65649711574556));
#21282=CARTESIAN_POINT('Origin',(0.,-1.9,7.));
#21283=CARTESIAN_POINT('',(-1.5,-1.8,7.));
#21284=CARTESIAN_POINT('Origin',(0.,-1.8,7.));
#21285=CARTESIAN_POINT('',(-1.5,1.8,7.));
#21286=CARTESIAN_POINT('',(-1.5,-1.9,7.));
#21287=CARTESIAN_POINT('Origin',(0.,1.8,7.));
#21288=CARTESIAN_POINT('Origin',(2.8,-1.,-0.1));
#21289=CARTESIAN_POINT('',(2.575,-1.,0.));
#21290=CARTESIAN_POINT('Origin',(2.8,-1.,0.));
#21291=CARTESIAN_POINT('',(2.575,-1.,0.8));
#21292=CARTESIAN_POINT('',(2.575,-1.,-0.1));
#21293=CARTESIAN_POINT('Origin',(2.8,-1.,0.8));
#21294=CARTESIAN_POINT('Origin',(-2.8,1.,-0.1));
#21295=CARTESIAN_POINT('',(-3.025,1.,0.));
#21296=CARTESIAN_POINT('Origin',(-2.8,1.,0.));
#21297=CARTESIAN_POINT('',(-3.025,1.,0.8));
#21298=CARTESIAN_POINT('',(-3.025,1.,-0.1));
#21299=CARTESIAN_POINT('Origin',(-2.8,1.,0.8));
#21300=CARTESIAN_POINT('Origin',(-2.8,-1.,-0.1));
#21301=CARTESIAN_POINT('',(-3.025,-1.,0.));
#21302=CARTESIAN_POINT('Origin',(-2.8,-1.,0.));
#21303=CARTESIAN_POINT('',(-3.025,-1.,0.8));
#21304=CARTESIAN_POINT('',(-3.025,-1.,-0.1));
#21305=CARTESIAN_POINT('Origin',(-2.8,-1.,0.8));
#21306=CARTESIAN_POINT('Origin',(2.8,1.,-0.1));
#21307=CARTESIAN_POINT('',(2.575,1.,0.));
#21308=CARTESIAN_POINT('Origin',(2.8,1.,0.));
#21309=CARTESIAN_POINT('',(2.575,1.,0.8));
#21310=CARTESIAN_POINT('',(2.575,1.,-0.1));
#21311=CARTESIAN_POINT('Origin',(2.8,1.,0.8));
#21312=CARTESIAN_POINT('Origin',(-3.4,-1.8,0.8));
#21313=CARTESIAN_POINT('',(2.2,-1.8,0.8));
#21314=CARTESIAN_POINT('',(2.2,1.8,0.8));
#21315=CARTESIAN_POINT('',(2.2,-1.8,0.8));
#21316=CARTESIAN_POINT('',(3.4,-1.8,0.8));
#21317=CARTESIAN_POINT('',(3.4,-1.8,0.8));
#21318=CARTESIAN_POINT('',(3.4,1.8,0.8));
#21319=CARTESIAN_POINT('',(3.4,-1.8,0.8));
#21320=CARTESIAN_POINT('',(3.4,1.8,0.8));
#21321=CARTESIAN_POINT('Origin',(-3.4,-1.8,0.8));
#21322=CARTESIAN_POINT('',(-2.2,1.8,0.8));
#21323=CARTESIAN_POINT('',(-2.2,-1.8,0.8));
#21324=CARTESIAN_POINT('',(-2.2,0.,0.8));
#21325=CARTESIAN_POINT('',(-3.4,1.8,0.8));
#21326=CARTESIAN_POINT('',(3.4,1.8,0.8));
#21327=CARTESIAN_POINT('',(-3.4,-1.8,0.8));
#21328=CARTESIAN_POINT('',(-3.4,-1.8,0.8));
#21329=CARTESIAN_POINT('',(3.4,-1.8,0.8));
#21330=CARTESIAN_POINT('Origin',(-3.4,-1.8,0.));
#21331=CARTESIAN_POINT('',(-3.4,-1.8,0.));
#21332=CARTESIAN_POINT('',(-3.4,-1.8,0.8));
#21333=CARTESIAN_POINT('',(-3.4,1.8,0.));
#21334=CARTESIAN_POINT('',(-3.4,1.8,0.8));
#21335=CARTESIAN_POINT('',(-3.4,-1.8,0.));
#21336=CARTESIAN_POINT('Origin',(3.4,-1.8,0.8));
#21337=CARTESIAN_POINT('',(3.4,-1.8,0.));
#21338=CARTESIAN_POINT('',(3.4,-1.8,0.));
#21339=CARTESIAN_POINT('',(3.4,1.8,0.));
#21340=CARTESIAN_POINT('',(3.4,-1.8,0.));
#21341=CARTESIAN_POINT('',(3.4,1.8,0.));
#21342=CARTESIAN_POINT('Origin',(-2.2,-1.8,0.));
#21343=CARTESIAN_POINT('',(2.2,-1.8,9.2));
#21344=CARTESIAN_POINT('',(2.2,-1.8,0.));
#21345=CARTESIAN_POINT('',(-2.2,-1.8,9.2));
#21346=CARTESIAN_POINT('',(-2.2,-1.8,9.2));
#21347=CARTESIAN_POINT('',(-2.2,-1.8,0.));
#21348=CARTESIAN_POINT('',(-3.4,-1.8,0.));
#21349=CARTESIAN_POINT('Origin',(2.2,-1.8,0.));
#21350=CARTESIAN_POINT('',(2.2,1.8,9.2));
#21351=CARTESIAN_POINT('',(2.2,1.8,0.));
#21352=CARTESIAN_POINT('',(2.2,-1.8,9.2));
#21353=CARTESIAN_POINT('Origin',(2.2,1.8,0.));
#21354=CARTESIAN_POINT('',(-2.2,1.8,9.2));
#21355=CARTESIAN_POINT('',(-2.2,1.8,0.));
#21356=CARTESIAN_POINT('',(2.2,1.8,9.2));
#21357=CARTESIAN_POINT('',(-3.4,1.8,0.));
#21358=CARTESIAN_POINT('Origin',(-2.2,1.8,0.));
#21359=CARTESIAN_POINT('',(-2.2,1.8,9.2));
#21360=CARTESIAN_POINT('Origin',(0.,0.,9.2));
#21361=CARTESIAN_POINT('Origin',(0.,0.,0.));
#26921=UNCERTAINTY_MEASURE_WITH_UNIT(LENGTH_MEASURE(0.001),#27070,
'DISTANCE_ACCURACY_VALUE',
'Maximum model space distance between geometric entities at asserted c
onnectivities');
#26992=UNCERTAINTY_MEASURE_WITH_UNIT(LENGTH_MEASURE(0.001),#27070,
'DISTANCE_ACCURACY_VALUE',
'Maximum model space distance between geometric entities at asserted c
onnectivities');
#26998=(
GEOMETRIC_REPRESENTATION_CONTEXT(3)
GLOBAL_UNCERTAINTY_ASSIGNED_CONTEXT((#26921))
GLOBAL_UNIT_ASSIGNED_CONTEXT((#27070,#27072,#27073))
REPRESENTATION_CONTEXT('','3D')
);
#27069=(
GEOMETRIC_REPRESENTATION_CONTEXT(3)
GLOBAL_UNCERTAINTY_ASSIGNED_CONTEXT((#26992))
GLOBAL_UNIT_ASSIGNED_CONTEXT((#27070,#27072,#27073))
REPRESENTATION_CONTEXT('','3D')
);
#27070=(
LENGTH_UNIT()
NAMED_UNIT(*)
SI_UNIT(.CENTI.,.METRE.)
);
#27072=(
NAMED_UNIT(*)
PLANE_ANGLE_UNIT()
SI_UNIT($,.RADIAN.)
);
#27073=(
NAMED_UNIT(*)
SI_UNIT($,.STERADIAN.)
SOLID_ANGLE_UNIT()
);
#27079=SHAPE_DEFINITION_REPRESENTATION(#27155,#27356);
#27155=PRODUCT_DEFINITION_SHAPE('',$,#27433);
#27356=SHAPE_REPRESENTATION('',(#14677),#26998);
#27427=PRODUCT_DEFINITION_CONTEXT('part definition',#27657,'design');
#27433=PRODUCT_DEFINITION('Fixed bearing block','Fixed bearing block',#27509,
#27427);
#27509=PRODUCT_DEFINITION_FORMATION('',$,#27664);
#27657=APPLICATION_CONTEXT(
'Core Data for Automotive Mechanical Design Process');
#27658=PRODUCT_CONTEXT('part definition',#27657,'mechanical');
#27664=PRODUCT('Fixed bearing block','Fixed bearing block',
'Fixed bearing block',(#27658));
#27791=COLOUR_RGB('Grey',0.48,0.52,0.57);
#27792=FILL_AREA_STYLE_COLOUR('',#27791);
#27793=FILL_AREA_STYLE('',(#27792));
#27794=SURFACE_STYLE_FILL_AREA(#27793);
#27795=SURFACE_SIDE_STYLE('',(#27794));
#27796=SURFACE_STYLE_USAGE(.BOTH.,#27795);
#27797=PRESENTATION_STYLE_ASSIGNMENT((#27796));
ENDSEC;
END-ISO-10303-21;
